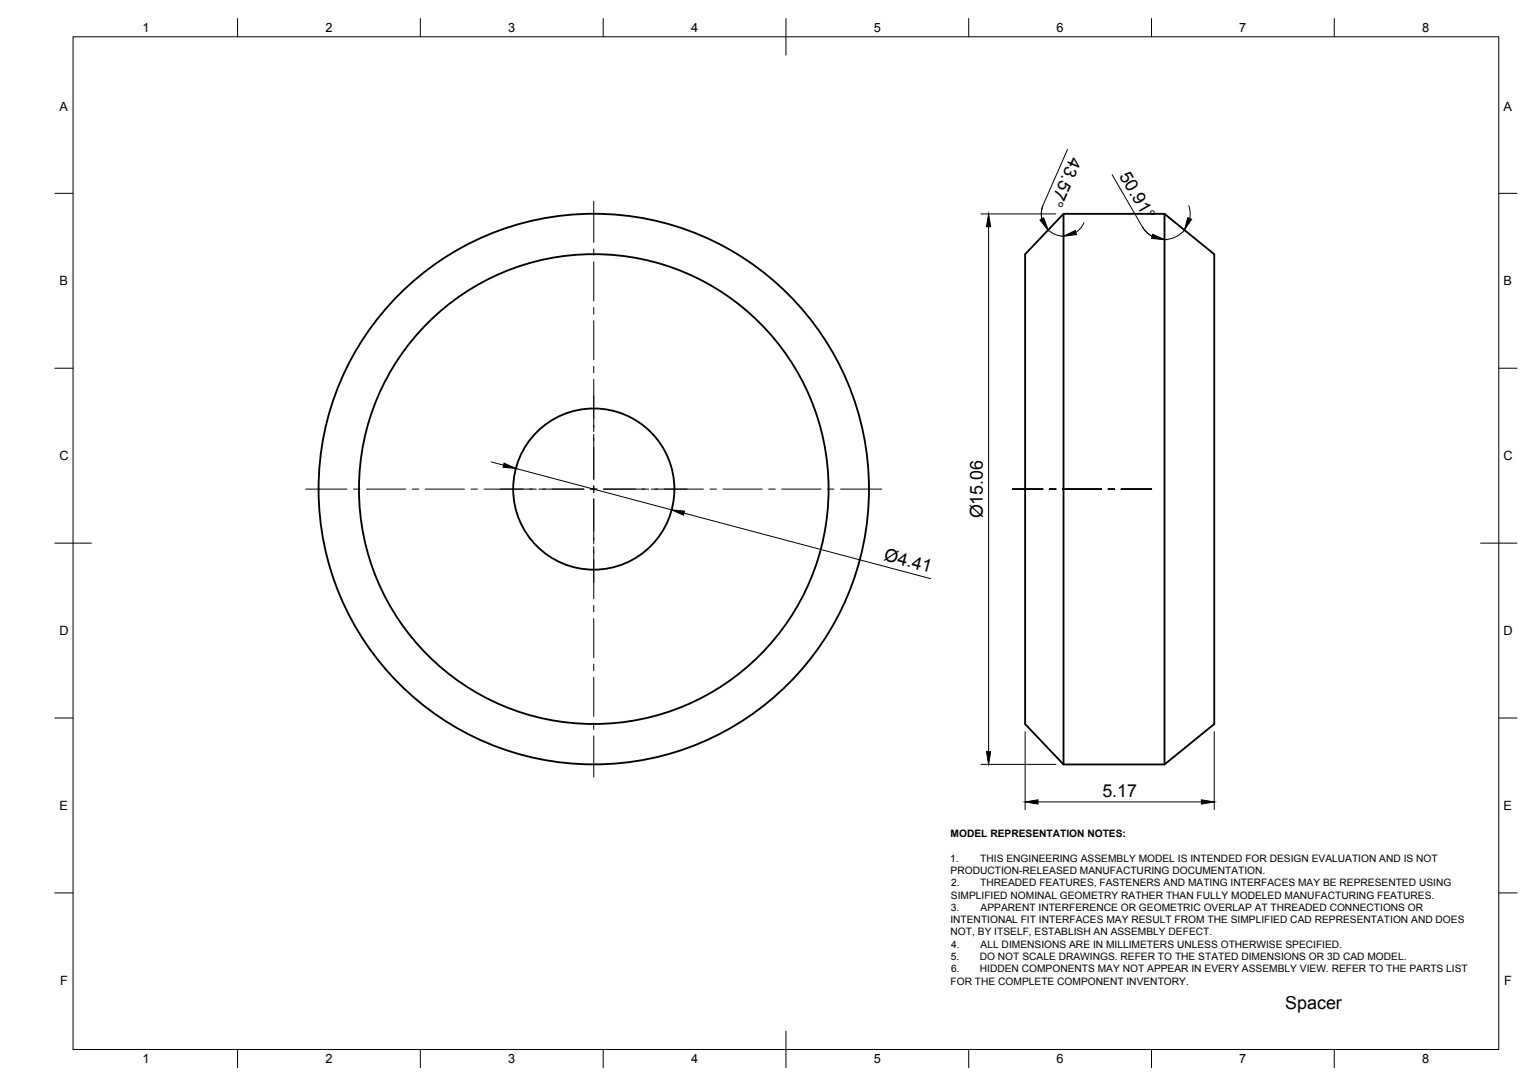
ISO-10303-21;
HEADER;
/* Generated by software containing ST-Developer
 * from STEP Tools, Inc. (www.steptools.com) 
 */

FILE_DESCRIPTION(
/* description */ (''),
/* implementation_level */ '2;1');

FILE_NAME(
/* name */ 'Spacer.step',
/* time_stamp */ '2026-10-06T13:05:37-07:00',
/* author */ (''),
/* organization */ (''),
/* preprocessor_version */ 'ST-DEVELOPER v20.2',
/* originating_system */ 'Autodesk Translation Framework v15.15.0.0',
/* authorisation */ '');

FILE_SCHEMA (('AUTOMOTIVE_DESIGN { 1 0 10303 214 3 1 1 }'));
ENDSEC;

DATA;
#10=MECHANICAL_DESIGN_GEOMETRIC_PRESENTATION_REPRESENTATION('',(#143),#28055);
#51=ORIENTED_CLOSED_SHELL('',*,#3684,.F.);
#52=ORIENTED_CLOSED_SHELL('',*,#3685,.F.);
#53=BREP_WITH_VOIDS('Body1',#3686,(#51,#52));
#114=TOROIDAL_SURFACE('',#4065,4.58180150972878,0.3);
#115=TOROIDAL_SURFACE('',#4067,4.58180150972878,0.3);
#123=SHAPE_REPRESENTATION_RELATIONSHIP('SRR','None',#28100,#133);
#133=ADVANCED_BREP_SHAPE_REPRESENTATION('',(#53),#28052);
#143=STYLED_ITEM('',(#28152),#53);
#171=CONICAL_SURFACE('',#4077,6.97561584944256,0.682200217168611);
#172=CONICAL_SURFACE('',#4083,6.97638033209901,0.810344007057193);
#197=FACE_BOUND('',#789,.T.);
#198=FACE_BOUND('',#793,.T.);
#199=FACE_BOUND('',#798,.T.);
#200=FACE_BOUND('',#802,.T.);
#242=PLANE('',#4063);
#243=PLANE('',#4071);
#244=PLANE('',#4080);
#245=PLANE('',#4085);
#361=CIRCLE('',#4061,4.88180150972878);
#362=CIRCLE('',#4062,4.88180150972878);
#363=CIRCLE('',#4064,4.58180150972878);
#364=CIRCLE('',#4066,0.3);
#365=CIRCLE('',#4068,4.58180150972878);
#366=CIRCLE('',#4069,0.3);
#367=CIRCLE('',#4070,4.88180150972878);
#368=CIRCLE('',#4072,4.88180150972878);
#369=CIRCLE('',#4075,2.204);
#370=CIRCLE('',#4076,2.204);
#371=CIRCLE('',#4078,7.52835105742136);
#372=CIRCLE('',#4079,6.42288064146375);
#373=CIRCLE('',#4082,7.52835105742136);
#374=CIRCLE('',#4084,6.42440960677665);
#557=FACE_OUTER_BOUND('',#787,.T.);
#558=FACE_OUTER_BOUND('',#788,.T.);
#559=FACE_OUTER_BOUND('',#790,.T.);
#560=FACE_OUTER_BOUND('',#791,.T.);
#561=FACE_OUTER_BOUND('',#792,.T.);
#562=FACE_OUTER_BOUND('',#794,.T.);
#563=FACE_OUTER_BOUND('',#795,.T.);
#564=FACE_OUTER_BOUND('',#796,.T.);
#565=FACE_OUTER_BOUND('',#797,.T.);
#566=FACE_OUTER_BOUND('',#799,.T.);
#567=FACE_OUTER_BOUND('',#800,.T.);
#568=FACE_OUTER_BOUND('',#801,.T.);
#787=EDGE_LOOP('',(#3282,#3283,#3284,#3285));
#788=EDGE_LOOP('',(#3286));
#789=EDGE_LOOP('',(#3287));
#790=EDGE_LOOP('',(#3288,#3289,#3290,#3291));
#791=EDGE_LOOP('',(#3292,#3293,#3294,#3295));
#792=EDGE_LOOP('',(#3296));
#793=EDGE_LOOP('',(#3297));
#794=EDGE_LOOP('',(#3298,#3299,#3300,#3301));
#795=EDGE_LOOP('',(#3302,#3303,#3304,#3305));
#796=EDGE_LOOP('',(#3306,#3307,#3308,#3309));
#797=EDGE_LOOP('',(#3310));
#798=EDGE_LOOP('',(#3311));
#799=EDGE_LOOP('',(#3312,#3313,#3314,#3315));
#800=EDGE_LOOP('',(#3316,#3317,#3318,#3319));
#801=EDGE_LOOP('',(#3320));
#802=EDGE_LOOP('',(#3321));
#951=LINE('',#25666,#1109);
#952=LINE('',#25683,#1110);
#953=LINE('',#25688,#1111);
#954=LINE('',#25694,#1112);
#955=LINE('',#25700,#1113);
#956=LINE('',#25703,#1114);
#1109=VECTOR('',#4768,4.88180150972878);
#1110=VECTOR('',#4793,4.88180150972878);
#1111=VECTOR('',#4798,2.204);
#1112=VECTOR('',#4805,6.97561584944256);
#1113=VECTOR('',#4814,7.52835105742136);
#1114=VECTOR('',#4817,6.97638033209901);
#1732=VERTEX_POINT('',#25663);
#1733=VERTEX_POINT('',#25665);
#1734=VERTEX_POINT('',#25669);
#1735=VERTEX_POINT('',#25674);
#1736=VERTEX_POINT('',#25676);
#1737=VERTEX_POINT('',#25680);
#1738=VERTEX_POINT('',#25685);
#1739=VERTEX_POINT('',#25687);
#1740=VERTEX_POINT('',#25691);
#1741=VERTEX_POINT('',#25693);
#1742=VERTEX_POINT('',#25698);
#1743=VERTEX_POINT('',#25702);
#2254=EDGE_CURVE('',#1732,#1732,#361,.T.);
#2255=EDGE_CURVE('',#1732,#1733,#951,.T.);
#2256=EDGE_CURVE('',#1733,#1733,#362,.T.);
#2257=EDGE_CURVE('',#1734,#1734,#363,.T.);
#2258=EDGE_CURVE('',#1733,#1734,#364,.T.);
#2259=EDGE_CURVE('',#1735,#1735,#365,.T.);
#2260=EDGE_CURVE('',#1735,#1736,#366,.T.);
#2261=EDGE_CURVE('',#1736,#1736,#367,.T.);
#2262=EDGE_CURVE('',#1737,#1737,#368,.T.);
#2263=EDGE_CURVE('',#1736,#1737,#952,.T.);
#2264=EDGE_CURVE('',#1738,#1738,#369,.T.);
#2265=EDGE_CURVE('',#1738,#1739,#953,.T.);
#2266=EDGE_CURVE('',#1739,#1739,#370,.T.);
#2267=EDGE_CURVE('',#1740,#1740,#371,.T.);
#2268=EDGE_CURVE('',#1740,#1741,#954,.T.);
#2269=EDGE_CURVE('',#1741,#1741,#372,.T.);
#2270=EDGE_CURVE('',#1742,#1742,#373,.T.);
#2271=EDGE_CURVE('',#1742,#1740,#955,.T.);
#2272=EDGE_CURVE('',#1742,#1743,#956,.T.);
#2273=EDGE_CURVE('',#1743,#1743,#374,.T.);
#3282=ORIENTED_EDGE('',*,*,#2254,.F.);
#3283=ORIENTED_EDGE('',*,*,#2255,.T.);
#3284=ORIENTED_EDGE('',*,*,#2256,.T.);
#3285=ORIENTED_EDGE('',*,*,#2255,.F.);
#3286=ORIENTED_EDGE('',*,*,#2254,.T.);
#3287=ORIENTED_EDGE('',*,*,#2257,.F.);
#3288=ORIENTED_EDGE('',*,*,#2256,.F.);
#3289=ORIENTED_EDGE('',*,*,#2258,.T.);
#3290=ORIENTED_EDGE('',*,*,#2257,.T.);
#3291=ORIENTED_EDGE('',*,*,#2258,.F.);
#3292=ORIENTED_EDGE('',*,*,#2259,.T.);
#3293=ORIENTED_EDGE('',*,*,#2260,.T.);
#3294=ORIENTED_EDGE('',*,*,#2261,.T.);
#3295=ORIENTED_EDGE('',*,*,#2260,.F.);
#3296=ORIENTED_EDGE('',*,*,#2262,.F.);
#3297=ORIENTED_EDGE('',*,*,#2259,.F.);
#3298=ORIENTED_EDGE('',*,*,#2261,.F.);
#3299=ORIENTED_EDGE('',*,*,#2263,.T.);
#3300=ORIENTED_EDGE('',*,*,#2262,.T.);
#3301=ORIENTED_EDGE('',*,*,#2263,.F.);
#3302=ORIENTED_EDGE('',*,*,#2264,.F.);
#3303=ORIENTED_EDGE('',*,*,#2265,.T.);
#3304=ORIENTED_EDGE('',*,*,#2266,.F.);
#3305=ORIENTED_EDGE('',*,*,#2265,.F.);
#3306=ORIENTED_EDGE('',*,*,#2267,.F.);
#3307=ORIENTED_EDGE('',*,*,#2268,.T.);
#3308=ORIENTED_EDGE('',*,*,#2269,.T.);
#3309=ORIENTED_EDGE('',*,*,#2268,.F.);
#3310=ORIENTED_EDGE('',*,*,#2269,.F.);
#3311=ORIENTED_EDGE('',*,*,#2264,.T.);
#3312=ORIENTED_EDGE('',*,*,#2270,.F.);
#3313=ORIENTED_EDGE('',*,*,#2271,.T.);
#3314=ORIENTED_EDGE('',*,*,#2267,.T.);
#3315=ORIENTED_EDGE('',*,*,#2271,.F.);
#3316=ORIENTED_EDGE('',*,*,#2270,.T.);
#3317=ORIENTED_EDGE('',*,*,#2272,.T.);
#3318=ORIENTED_EDGE('',*,*,#2273,.F.);
#3319=ORIENTED_EDGE('',*,*,#2272,.F.);
#3320=ORIENTED_EDGE('',*,*,#2273,.T.);
#3321=ORIENTED_EDGE('',*,*,#2266,.T.);
#3465=CYLINDRICAL_SURFACE('',#4060,4.88180150972878);
#3466=CYLINDRICAL_SURFACE('',#4073,4.88180150972878);
#3467=CYLINDRICAL_SURFACE('',#4074,2.204);
#3468=CYLINDRICAL_SURFACE('',#4081,7.52835105742136);
#3649=ADVANCED_FACE('',(#557),#3465,.F.);
#3650=ADVANCED_FACE('',(#558,#197),#242,.T.);
#3651=ADVANCED_FACE('',(#559),#114,.T.);
#3652=ADVANCED_FACE('',(#560),#115,.T.);
#3653=ADVANCED_FACE('',(#561,#198),#243,.T.);
#3654=ADVANCED_FACE('',(#562),#3466,.F.);
#3655=ADVANCED_FACE('',(#563),#3467,.F.);
#3656=ADVANCED_FACE('',(#564),#171,.T.);
#3657=ADVANCED_FACE('',(#565,#199),#244,.T.);
#3658=ADVANCED_FACE('',(#566),#3468,.T.);
#3659=ADVANCED_FACE('',(#567),#172,.T.);
#3660=ADVANCED_FACE('',(#568,#200),#245,.T.);
#3684=CLOSED_SHELL('',(#3649,#3650,#3651));
#3685=CLOSED_SHELL('',(#3652,#3653,#3654));
#3686=CLOSED_SHELL('',(#3655,#3656,#3657,#3658,#3659,#3660));
#4059=AXIS2_PLACEMENT_3D('',#25661,#4762,#4763);
#4060=AXIS2_PLACEMENT_3D('',#25662,#4764,#4765);
#4061=AXIS2_PLACEMENT_3D('',#25664,#4766,#4767);
#4062=AXIS2_PLACEMENT_3D('',#25667,#4769,#4770);
#4063=AXIS2_PLACEMENT_3D('',#25668,#4771,#4772);
#4064=AXIS2_PLACEMENT_3D('',#25670,#4773,#4774);
#4065=AXIS2_PLACEMENT_3D('',#25671,#4775,#4776);
#4066=AXIS2_PLACEMENT_3D('',#25672,#4777,#4778);
#4067=AXIS2_PLACEMENT_3D('',#25673,#4779,#4780);
#4068=AXIS2_PLACEMENT_3D('',#25675,#4781,#4782);
#4069=AXIS2_PLACEMENT_3D('',#25677,#4783,#4784);
#4070=AXIS2_PLACEMENT_3D('',#25678,#4785,#4786);
#4071=AXIS2_PLACEMENT_3D('',#25679,#4787,#4788);
#4072=AXIS2_PLACEMENT_3D('',#25681,#4789,#4790);
#4073=AXIS2_PLACEMENT_3D('',#25682,#4791,#4792);
#4074=AXIS2_PLACEMENT_3D('',#25684,#4794,#4795);
#4075=AXIS2_PLACEMENT_3D('',#25686,#4796,#4797);
#4076=AXIS2_PLACEMENT_3D('',#25689,#4799,#4800);
#4077=AXIS2_PLACEMENT_3D('',#25690,#4801,#4802);
#4078=AXIS2_PLACEMENT_3D('',#25692,#4803,#4804);
#4079=AXIS2_PLACEMENT_3D('',#25695,#4806,#4807);
#4080=AXIS2_PLACEMENT_3D('',#25696,#4808,#4809);
#4081=AXIS2_PLACEMENT_3D('',#25697,#4810,#4811);
#4082=AXIS2_PLACEMENT_3D('',#25699,#4812,#4813);
#4083=AXIS2_PLACEMENT_3D('',#25701,#4815,#4816);
#4084=AXIS2_PLACEMENT_3D('',#25704,#4818,#4819);
#4085=AXIS2_PLACEMENT_3D('',#25705,#4820,#4821);
#4762=DIRECTION('axis',(0.,0.,1.));
#4763=DIRECTION('refdir',(1.,0.,0.));
#4764=DIRECTION('center_axis',(1.,0.,0.));
#4765=DIRECTION('ref_axis',(0.,0.,-1.));
#4766=DIRECTION('center_axis',(1.,0.,0.));
#4767=DIRECTION('ref_axis',(0.,0.,-1.));
#4768=DIRECTION('',(1.,0.,0.));
#4769=DIRECTION('center_axis',(1.,0.,0.));
#4770=DIRECTION('ref_axis',(0.,0.,-1.));
#4771=DIRECTION('center_axis',(1.,0.,0.));
#4772=DIRECTION('ref_axis',(0.,0.,-1.));
#4773=DIRECTION('center_axis',(1.,0.,0.));
#4774=DIRECTION('ref_axis',(0.,0.,-1.));
#4775=DIRECTION('center_axis',(1.,0.,0.));
#4776=DIRECTION('ref_axis',(0.,0.,-1.));
#4777=DIRECTION('center_axis',(0.,-1.,-1.22464679914735E-16));
#4778=DIRECTION('ref_axis',(0.,-1.22464679914735E-16,1.));
#4779=DIRECTION('center_axis',(1.,0.,0.));
#4780=DIRECTION('ref_axis',(0.,0.,-1.));
#4781=DIRECTION('center_axis',(-1.,0.,0.));
#4782=DIRECTION('ref_axis',(0.,0.,-1.));
#4783=DIRECTION('center_axis',(0.,-1.,-1.22464679914735E-16));
#4784=DIRECTION('ref_axis',(0.,-1.22464679914735E-16,1.));
#4785=DIRECTION('center_axis',(1.,0.,0.));
#4786=DIRECTION('ref_axis',(0.,0.,-1.));
#4787=DIRECTION('center_axis',(-1.,0.,0.));
#4788=DIRECTION('ref_axis',(0.,0.,1.));
#4789=DIRECTION('center_axis',(1.,0.,0.));
#4790=DIRECTION('ref_axis',(0.,0.,-1.));
#4791=DIRECTION('center_axis',(1.,0.,0.));
#4792=DIRECTION('ref_axis',(0.,0.,-1.));
#4793=DIRECTION('',(1.,0.,0.));
#4794=DIRECTION('center_axis',(1.,0.,0.));
#4795=DIRECTION('ref_axis',(0.,0.,-1.));
#4796=DIRECTION('center_axis',(1.,0.,0.));
#4797=DIRECTION('ref_axis',(0.,0.,-1.));
#4798=DIRECTION('',(1.,0.,0.));
#4799=DIRECTION('center_axis',(-1.,0.,0.));
#4800=DIRECTION('ref_axis',(0.,0.,-1.));
#4801=DIRECTION('center_axis',(1.,0.,0.));
#4802=DIRECTION('ref_axis',(0.,0.,-1.));
#4803=DIRECTION('center_axis',(1.,0.,0.));
#4804=DIRECTION('ref_axis',(0.,0.,-1.));
#4805=DIRECTION('',(-0.776187356563468,7.72142659683039E-17,-0.630502329504829));
#4806=DIRECTION('center_axis',(1.,0.,0.));
#4807=DIRECTION('ref_axis',(0.,0.,-1.));
#4808=DIRECTION('center_axis',(-1.,0.,0.));
#4809=DIRECTION('ref_axis',(0.,0.,1.));
#4810=DIRECTION('center_axis',(1.,0.,0.));
#4811=DIRECTION('ref_axis',(0.,0.,-1.));
#4812=DIRECTION('center_axis',(1.,0.,0.));
#4813=DIRECTION('ref_axis',(0.,0.,-1.));
#4814=DIRECTION('',(-1.,0.,0.));
#4815=DIRECTION('center_axis',(-1.,0.,0.));
#4816=DIRECTION('ref_axis',(0.,0.,-1.));
#4817=DIRECTION('',(0.689249232259327,-8.87286394090086E-17,-0.724524323835942));
#4818=DIRECTION('center_axis',(1.,0.,0.));
#4819=DIRECTION('ref_axis',(0.,0.,-1.));
#4820=DIRECTION('center_axis',(1.,0.,0.));
#4821=DIRECTION('ref_axis',(0.,0.,-1.));
#25661=CARTESIAN_POINT('',(0.,0.,0.));
#25662=CARTESIAN_POINT('Origin',(78.8794814490059,0.,0.));
#25663=CARTESIAN_POINT('',(77.4376255944759,-5.97848259296207E-16,4.88180150972878));
#25664=CARTESIAN_POINT('Origin',(77.4376255944759,0.,0.));
#25665=CARTESIAN_POINT('',(77.7376255944759,-5.97848259296207E-16,4.88180150972878));
#25666=CARTESIAN_POINT('',(78.8794814490059,-5.97848259296207E-16,4.88180150972878));
#25667=CARTESIAN_POINT('Origin',(77.7376255944759,0.,0.));
#25668=CARTESIAN_POINT('Origin',(77.4376255944759,0.,0.));
#25669=CARTESIAN_POINT('',(77.4376255944759,-5.61108855321787E-16,4.58180150972878));
#25670=CARTESIAN_POINT('Origin',(77.4376255944759,0.,0.));
#25671=CARTESIAN_POINT('Origin',(77.7376255944759,0.,0.));
#25672=CARTESIAN_POINT('Origin',(77.7376255944759,-5.61108855321786E-16,
4.58180150972878));
#25673=CARTESIAN_POINT('Origin',(80.0213373035359,0.,0.));
#25674=CARTESIAN_POINT('',(80.3213373035359,-5.61108855321787E-16,4.58180150972878));
#25675=CARTESIAN_POINT('Origin',(80.3213373035359,0.,0.));
#25676=CARTESIAN_POINT('',(80.0213373035359,-5.97848259296207E-16,4.88180150972878));
#25677=CARTESIAN_POINT('Origin',(80.0213373035359,-5.61108855321786E-16,
4.58180150972878));
#25678=CARTESIAN_POINT('Origin',(80.0213373035359,0.,0.));
#25679=CARTESIAN_POINT('Origin',(80.3213373035359,0.,-4.88180150972878));
#25680=CARTESIAN_POINT('',(80.3213373035359,-5.97848259296207E-16,4.88180150972878));
#25681=CARTESIAN_POINT('Origin',(80.3213373035359,0.,0.));
#25682=CARTESIAN_POINT('Origin',(78.8794814490059,0.,0.));
#25683=CARTESIAN_POINT('',(78.8794814490059,-5.97848259296207E-16,4.88180150972878));
#25684=CARTESIAN_POINT('Origin',(66.9212607628943,0.,0.));
#25685=CARTESIAN_POINT('',(76.270750134144,-2.69912154532077E-16,2.204));
#25686=CARTESIAN_POINT('Origin',(76.270750134144,0.,0.));
#25687=CARTESIAN_POINT('',(81.4430005297901,2.69912154532077E-16,2.204));
#25688=CARTESIAN_POINT('',(66.9212607628943,-2.69912154532077E-16,2.204));
#25689=CARTESIAN_POINT('Origin',(81.4430005297901,0.,0.));
#25690=CARTESIAN_POINT('Origin',(76.951201355153,0.,0.));
#25691=CARTESIAN_POINT('',(77.6316525761621,-9.21957102532866E-16,7.52835105742136));
#25692=CARTESIAN_POINT('Origin',(77.6316525761621,0.,0.));
#25693=CARTESIAN_POINT('',(76.270750134144,-7.86576021887409E-16,6.42288064146376));
#25694=CARTESIAN_POINT('',(76.951201355153,-8.54266562210138E-16,6.97561584944256));
#25695=CARTESIAN_POINT('Origin',(76.270750134144,0.,0.));
#25696=CARTESIAN_POINT('Origin',(76.270750134144,0.,-6.42288064146375));
#25697=CARTESIAN_POINT('Origin',(79.0122297603055,0.,0.));
#25698=CARTESIAN_POINT('',(80.392806944449,-9.21957102532866E-16,7.52835105742136));
#25699=CARTESIAN_POINT('Origin',(80.392806944449,0.,0.));
#25700=CARTESIAN_POINT('',(79.0122297603055,-9.21957102532866E-16,7.52835105742136));
#25701=CARTESIAN_POINT('Origin',(80.9179037371196,0.,0.));
#25702=CARTESIAN_POINT('',(81.4430005297901,-7.86763266135053E-16,6.42440960677665));
#25703=CARTESIAN_POINT('',(80.9179037371196,8.5436018433396E-16,6.97638033209901));
#25704=CARTESIAN_POINT('Origin',(81.4430005297901,0.,0.));
#25705=CARTESIAN_POINT('Origin',(81.4430005297901,0.,0.));
#28040=UNCERTAINTY_MEASURE_WITH_UNIT(LENGTH_MEASURE(0.01),#28056,
'DISTANCE_ACCURACY_VALUE',
'Maximum model space distance between geometric entities at asserted c
onnectivities');
#28043=UNCERTAINTY_MEASURE_WITH_UNIT(LENGTH_MEASURE(0.01),#28056,
'DISTANCE_ACCURACY_VALUE',
'Maximum model space distance between geometric entities at asserted c
onnectivities');
#28052=(
GEOMETRIC_REPRESENTATION_CONTEXT(3)
GLOBAL_UNCERTAINTY_ASSIGNED_CONTEXT((#28040))
GLOBAL_UNIT_ASSIGNED_CONTEXT((#28056,#28058,#28059))
REPRESENTATION_CONTEXT('','3D')
);
#28055=(
GEOMETRIC_REPRESENTATION_CONTEXT(3)
GLOBAL_UNCERTAINTY_ASSIGNED_CONTEXT((#28043))
GLOBAL_UNIT_ASSIGNED_CONTEXT((#28056,#28058,#28059))
REPRESENTATION_CONTEXT('','3D')
);
#28056=(
LENGTH_UNIT()
NAMED_UNIT(*)
SI_UNIT(.MILLI.,.METRE.)
);
#28058=(
NAMED_UNIT(*)
PLANE_ANGLE_UNIT()
SI_UNIT($,.RADIAN.)
);
#28059=(
NAMED_UNIT(*)
SI_UNIT($,.STERADIAN.)
SOLID_ANGLE_UNIT()
);
#28068=SHAPE_DEFINITION_REPRESENTATION(#28079,#28100);
#28079=PRODUCT_DEFINITION_SHAPE('',$,#28112);
#28100=SHAPE_REPRESENTATION('',(#4059),#28052);
#28103=PRODUCT_DEFINITION_CONTEXT('part definition',#28138,'design');
#28112=PRODUCT_DEFINITION('spacer','Spacer',#28123,#28103);
#28123=PRODUCT_DEFINITION_FORMATION('',$,#28148);
#28138=APPLICATION_CONTEXT(
'Core Data for Automotive Mechanical Design Process');
#28139=PRODUCT_CONTEXT('part definition',#28138,'mechanical');
#28148=PRODUCT('spacer','Spacer',$,(#28139));
#28152=PRESENTATION_STYLE_ASSIGNMENT((#28155));
#28155=SURFACE_STYLE_USAGE(.BOTH.,#28158);
#28158=SURFACE_SIDE_STYLE('',(#28161));
#28161=SURFACE_STYLE_FILL_AREA(#28164);
#28164=FILL_AREA_STYLE('Opaque(160,160,160)',(#28167));
#28167=FILL_AREA_STYLE_COLOUR('Opaque(160,160,160)',#28170);
#28170=COLOUR_RGB('Opaque(160,160,160)', 0.66274510, 0.83137255, 0.94901961);
ENDSEC;
END-ISO-10303-21;
